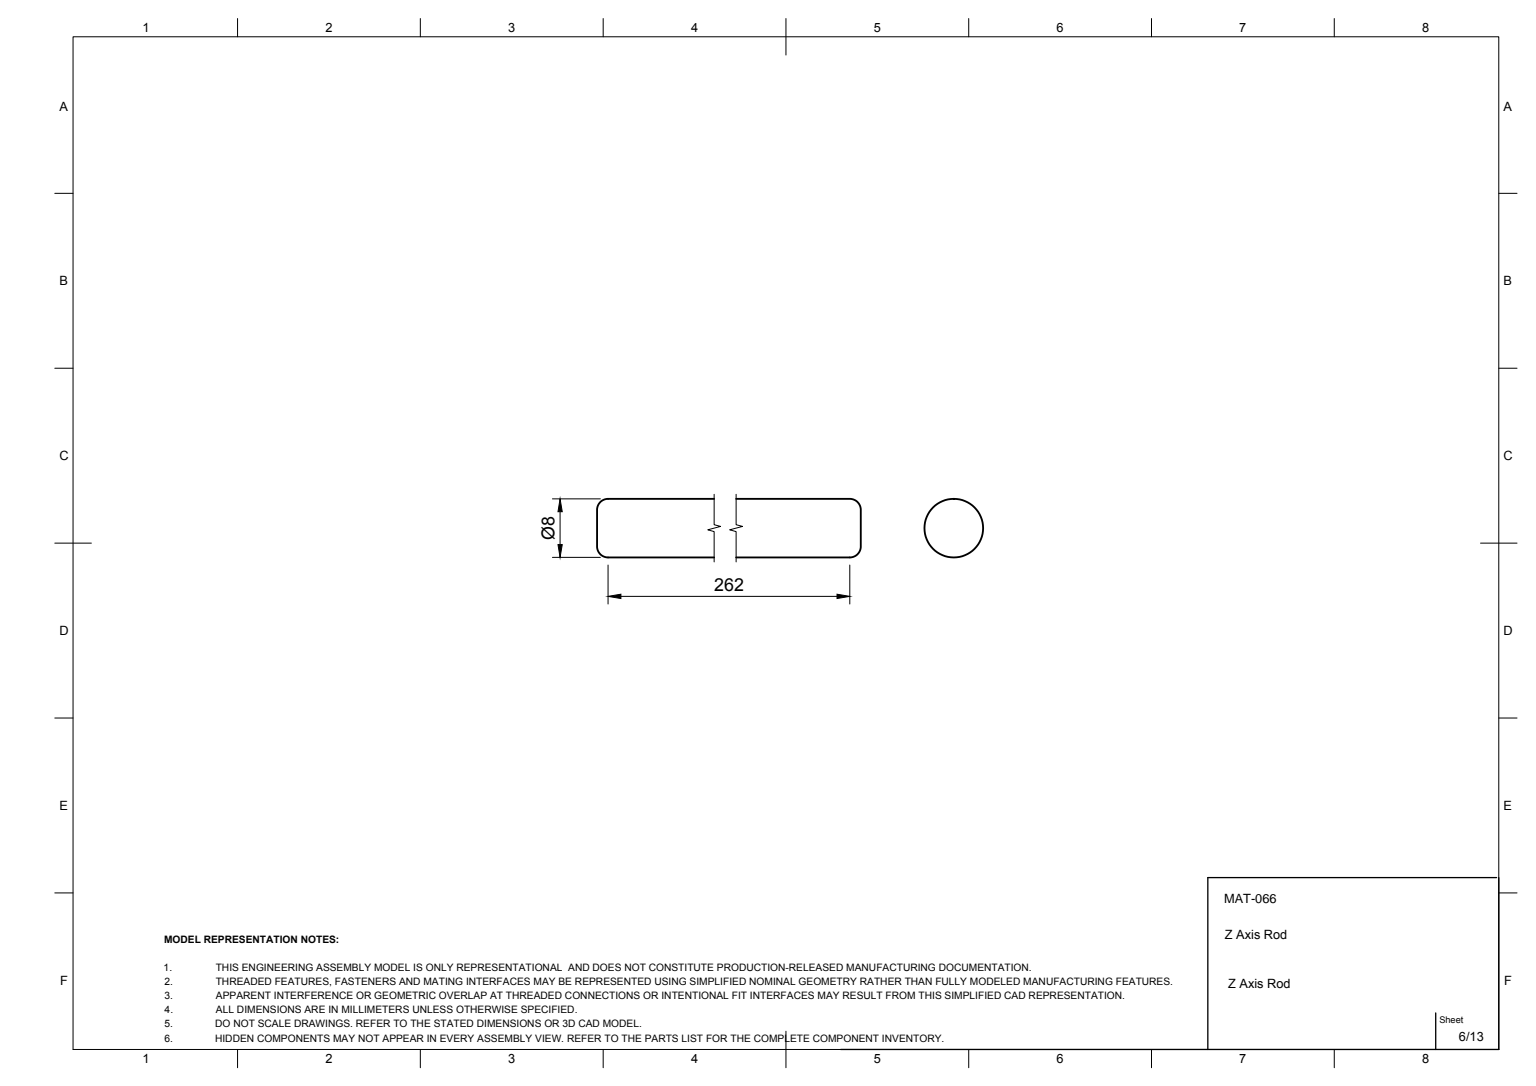
ISO-10303-21;
HEADER;
/* Generated by software containing ST-Developer
 * from STEP Tools, Inc. (www.steptools.com) 
 */

FILE_DESCRIPTION(
/* description */ ('CAx-IF Rec.Pracs.---Representation and Presentation of Product Manufa
cturing Information (PMI)---4.0---2014-10-13'),
/* implementation_level */ '2;1');

FILE_NAME(
/* name */ 'Z Axis Rod.step',
/* time_stamp */ '2026-10-24T15:58:00-07:00',
/* author */ (''),
/* organization */ (''),
/* preprocessor_version */ 'ST-DEVELOPER v20.2',
/* originating_system */ 'Autodesk Translation Framework v15.17.0.0',
/* authorisation */ '');

FILE_SCHEMA (('AP242_MANAGED_MODEL_BASED_3D_ENGINEERING_MIM_LF { 1 0 10303 442 2 1 4 }'));
ENDSEC;

DATA;
#10=MECHANICAL_DESIGN_GEOMETRIC_PRESENTATION_REPRESENTATION('',(#132),#8944);
#109=TOROIDAL_SURFACE('',#5681,0.0025,0.0015);
#110=TOROIDAL_SURFACE('',#5683,0.0025,0.0015);
#114=SHAPE_REPRESENTATION_RELATIONSHIP('SRR','None',#8996,#123);
#123=ADVANCED_BREP_SHAPE_REPRESENTATION('',(#141),#8937);
#132=STYLED_ITEM('',(#9055),#141);
#141=MANIFOLD_SOLID_BREP('Body1',#5153);
#217=CYLINDRICAL_SURFACE('',#5672,0.004);
#522=FACE_OUTER_BOUND('',#841,.T.);
#523=FACE_OUTER_BOUND('',#842,.T.);
#524=FACE_OUTER_BOUND('',#843,.T.);
#525=FACE_OUTER_BOUND('',#844,.T.);
#526=FACE_OUTER_BOUND('',#845,.T.);
#841=EDGE_LOOP('',(#4523,#4524,#4525,#4526,#4527,#4528));
#842=EDGE_LOOP('',(#4529));
#843=EDGE_LOOP('',(#4530));
#844=EDGE_LOOP('',(#4531,#4532,#4533,#4534,#4535));
#845=EDGE_LOOP('',(#4536,#4537,#4538,#4539,#4540));
#1110=CIRCLE('',#5673,0.004);
#1111=CIRCLE('',#5674,0.004);
#1112=CIRCLE('',#5675,0.004);
#1113=CIRCLE('',#5676,0.004);
#1114=CIRCLE('',#5678,0.0025);
#1115=CIRCLE('',#5680,0.0025);
#1116=CIRCLE('',#5682,0.0015);
#1117=CIRCLE('',#5684,0.0015);
#1596=LINE('',#8690,#2051);
#2051=VECTOR('',#7071,0.004);
#2498=VERTEX_POINT('',#8686);
#2499=VERTEX_POINT('',#8687);
#2500=VERTEX_POINT('',#8689);
#2501=VERTEX_POINT('',#8691);
#2502=VERTEX_POINT('',#8696);
#2503=VERTEX_POINT('',#8699);
#3182=EDGE_CURVE('',#2498,#2499,#1110,.T.);
#3183=EDGE_CURVE('',#2499,#2500,#1596,.T.);
#3184=EDGE_CURVE('',#2500,#2501,#1111,.F.);
#3185=EDGE_CURVE('',#2501,#2500,#1112,.F.);
#3186=EDGE_CURVE('',#2499,#2498,#1113,.T.);
#3187=EDGE_CURVE('',#2502,#2502,#1114,.T.);
#3188=EDGE_CURVE('',#2503,#2503,#1115,.F.);
#3189=EDGE_CURVE('',#2498,#2503,#1116,.T.);
#3190=EDGE_CURVE('',#2502,#2501,#1117,.T.);
#4523=ORIENTED_EDGE('',*,*,#3182,.T.);
#4524=ORIENTED_EDGE('',*,*,#3183,.T.);
#4525=ORIENTED_EDGE('',*,*,#3184,.T.);
#4526=ORIENTED_EDGE('',*,*,#3185,.T.);
#4527=ORIENTED_EDGE('',*,*,#3183,.F.);
#4528=ORIENTED_EDGE('',*,*,#3186,.T.);
#4529=ORIENTED_EDGE('',*,*,#3187,.T.);
#4530=ORIENTED_EDGE('',*,*,#3188,.T.);
#4531=ORIENTED_EDGE('',*,*,#3182,.F.);
#4532=ORIENTED_EDGE('',*,*,#3189,.T.);
#4533=ORIENTED_EDGE('',*,*,#3188,.F.);
#4534=ORIENTED_EDGE('',*,*,#3189,.F.);
#4535=ORIENTED_EDGE('',*,*,#3186,.F.);
#4536=ORIENTED_EDGE('',*,*,#3187,.F.);
#4537=ORIENTED_EDGE('',*,*,#3190,.T.);
#4538=ORIENTED_EDGE('',*,*,#3184,.F.);
#4539=ORIENTED_EDGE('',*,*,#3185,.F.);
#4540=ORIENTED_EDGE('',*,*,#3190,.F.);
#4859=PLANE('',#5677);
#4860=PLANE('',#5679);
#5095=ADVANCED_FACE('',(#522),#217,.T.);
#5096=ADVANCED_FACE('',(#523),#4859,.T.);
#5097=ADVANCED_FACE('',(#524),#4860,.F.);
#5098=ADVANCED_FACE('',(#525),#109,.T.);
#5099=ADVANCED_FACE('',(#526),#110,.T.);
#5153=CLOSED_SHELL('',(#5095,#5096,#5097,#5098,#5099));
#5671=AXIS2_PLACEMENT_3D('',#8684,#7065,#7066);
#5672=AXIS2_PLACEMENT_3D('',#8685,#7067,#7068);
#5673=AXIS2_PLACEMENT_3D('',#8688,#7069,#7070);
#5674=AXIS2_PLACEMENT_3D('',#8692,#7072,#7073);
#5675=AXIS2_PLACEMENT_3D('',#8693,#7074,#7075);
#5676=AXIS2_PLACEMENT_3D('',#8694,#7076,#7077);
#5677=AXIS2_PLACEMENT_3D('',#8695,#7078,#7079);
#5678=AXIS2_PLACEMENT_3D('',#8697,#7080,#7081);
#5679=AXIS2_PLACEMENT_3D('',#8698,#7082,#7083);
#5680=AXIS2_PLACEMENT_3D('',#8700,#7084,#7085);
#5681=AXIS2_PLACEMENT_3D('',#8701,#7086,#7087);
#5682=AXIS2_PLACEMENT_3D('',#8702,#7088,#7089);
#5683=AXIS2_PLACEMENT_3D('',#8703,#7090,#7091);
#5684=AXIS2_PLACEMENT_3D('',#8704,#7092,#7093);
#7065=DIRECTION('axis',(0.,0.,1.));
#7066=DIRECTION('refdir',(1.,0.,0.));
#7067=DIRECTION('center_axis',(0.,0.,-1.));
#7068=DIRECTION('ref_axis',(-1.,0.,0.));
#7069=DIRECTION('center_axis',(0.,0.,1.));
#7070=DIRECTION('ref_axis',(1.,0.,0.));
#7071=DIRECTION('',(0.,0.,1.));
#7072=DIRECTION('center_axis',(0.,0.,1.));
#7073=DIRECTION('ref_axis',(1.,0.,0.));
#7074=DIRECTION('center_axis',(0.,0.,1.));
#7075=DIRECTION('ref_axis',(1.,0.,0.));
#7076=DIRECTION('center_axis',(0.,0.,1.));
#7077=DIRECTION('ref_axis',(1.,0.,0.));
#7078=DIRECTION('center_axis',(0.,0.,1.));
#7079=DIRECTION('ref_axis',(1.,0.,0.));
#7080=DIRECTION('center_axis',(0.,0.,1.));
#7081=DIRECTION('ref_axis',(1.,0.,0.));
#7082=DIRECTION('center_axis',(0.,0.,1.));
#7083=DIRECTION('ref_axis',(1.,0.,0.));
#7084=DIRECTION('center_axis',(0.,0.,1.));
#7085=DIRECTION('ref_axis',(1.,0.,0.));
#7086=DIRECTION('center_axis',(0.,0.,1.));
#7087=DIRECTION('ref_axis',(1.,0.,0.));
#7088=DIRECTION('center_axis',(1.22464679914735E-16,-1.,0.));
#7089=DIRECTION('ref_axis',(-1.,-1.22464679914735E-16,0.));
#7090=DIRECTION('center_axis',(0.,0.,1.));
#7091=DIRECTION('ref_axis',(1.,0.,0.));
#7092=DIRECTION('center_axis',(1.22464679914735E-16,-1.,0.));
#7093=DIRECTION('ref_axis',(-1.,-1.22464679914735E-16,0.));
#8684=CARTESIAN_POINT('',(0.,0.,0.));
#8685=CARTESIAN_POINT('Origin',(0.,2.4492935982947E-19,0.265));
#8686=CARTESIAN_POINT('',(-0.004,-2.44929359829471E-19,0.0015));
#8687=CARTESIAN_POINT('',(0.004,-2.44929359829471E-19,0.00149999999999999));
#8688=CARTESIAN_POINT('Origin',(0.,2.4492935982947E-19,0.0015));
#8689=CARTESIAN_POINT('',(0.004,-2.44929359829471E-19,0.2635));
#8690=CARTESIAN_POINT('',(0.004,-2.44929359829471E-19,0.265));
#8691=CARTESIAN_POINT('',(-0.004,-2.44929359829471E-19,0.2635));
#8692=CARTESIAN_POINT('Origin',(0.,2.4492935982947E-19,0.2635));
#8693=CARTESIAN_POINT('Origin',(0.,2.4492935982947E-19,0.2635));
#8694=CARTESIAN_POINT('Origin',(0.,2.4492935982947E-19,0.0015));
#8695=CARTESIAN_POINT('Origin',(0.,0.,0.265));
#8696=CARTESIAN_POINT('',(-0.0025,-6.12323399573683E-20,0.265));
#8697=CARTESIAN_POINT('Origin',(0.,2.4492935982947E-19,0.265));
#8698=CARTESIAN_POINT('Origin',(0.,0.,0.));
#8699=CARTESIAN_POINT('',(-0.0025,-6.12323399573683E-20,0.));
#8700=CARTESIAN_POINT('Origin',(0.,2.4492935982947E-19,0.));
#8701=CARTESIAN_POINT('Origin',(0.,2.4492935982947E-19,0.0015));
#8702=CARTESIAN_POINT('Origin',(-0.0025,-6.12323399573683E-20,0.0015));
#8703=CARTESIAN_POINT('Origin',(0.,2.4492935982947E-19,0.2635));
#8704=CARTESIAN_POINT('Origin',(-0.0025,-6.12323399573683E-20,0.2635));
#8925=UNCERTAINTY_MEASURE_WITH_UNIT(LENGTH_MEASURE(1.E-5),#8945,
'DISTANCE_ACCURACY_VALUE',
'Maximum model space distance between geometric entities at asserted c
onnectivities');
#8932=UNCERTAINTY_MEASURE_WITH_UNIT(LENGTH_MEASURE(1.E-5),#8945,
'DISTANCE_ACCURACY_VALUE',
'Maximum model space distance between geometric entities at asserted c
onnectivities');
#8937=(
GEOMETRIC_REPRESENTATION_CONTEXT(3)
GLOBAL_UNCERTAINTY_ASSIGNED_CONTEXT((#8925))
GLOBAL_UNIT_ASSIGNED_CONTEXT((#8945,#8946,#8947))
REPRESENTATION_CONTEXT('','3D')
);
#8944=(
GEOMETRIC_REPRESENTATION_CONTEXT(3)
GLOBAL_UNCERTAINTY_ASSIGNED_CONTEXT((#8932))
GLOBAL_UNIT_ASSIGNED_CONTEXT((#8945,#8946,#8947))
REPRESENTATION_CONTEXT('','3D')
);
#8945=(
LENGTH_UNIT()
NAMED_UNIT(*)
SI_UNIT($,.METRE.)
);
#8946=(
NAMED_UNIT(*)
PLANE_ANGLE_UNIT()
SI_UNIT($,.RADIAN.)
);
#8947=(
NAMED_UNIT(*)
SI_UNIT($,.STERADIAN.)
SOLID_ANGLE_UNIT()
);
#8952=SHAPE_DEFINITION_REPRESENTATION(#8963,#8996);
#8963=PRODUCT_DEFINITION_SHAPE('',$,#9008);
#8996=SHAPE_REPRESENTATION('',(#5671),#8937);
#9003=PRODUCT_DEFINITION_CONTEXT('part definition',#9038,'design');
#9008=PRODUCT_DEFINITION('Z Axis Rod','Z Axis Rod',#9019,#9003);
#9019=PRODUCT_DEFINITION_FORMATION('',$,#9044);
#9038=APPLICATION_CONTEXT('Managed model based 3d engineering');
#9039=PRODUCT_CONTEXT('part definition',#9038,'mechanical');
#9044=PRODUCT('Z Axis Rod','Z Axis Rod',
'LEGAL AND USAGE DISCLAIMER: this Data/Model is provided \X2\201C\X0\A
S IS\X2\201D\X0\ for informational and representational only. It is a 
geometric approximation and is NOT engineered, certified, or guarantee
d for dimensional accuracy, exact tolerances, or production-level prec
ision. Vendor disclaims all implied warranties including fitness for a
 particular purpose. DO NOT USE FOR DIRECT PHYSICAL MANUFACTURING, AUT
OMATED PRODUCTION, OR SAFETY-CRITICAL SYSTEMS without independent engi
neering verification and resolution of any design discrepancies.',(#9039));
#9055=PRESENTATION_STYLE_ASSIGNMENT((#9060));
#9060=SURFACE_STYLE_USAGE(.BOTH.,#9065);
#9065=SURFACE_SIDE_STYLE('',(#9070));
#9070=SURFACE_STYLE_FILL_AREA(#9075);
#9075=FILL_AREA_STYLE('Opaque(48,59,150)',(#9080));
#9080=FILL_AREA_STYLE_COLOUR('Opaque(48,59,150)',#9085);
#9085=COLOUR_RGB('Opaque(48,59,150)',0.188235294117647,0.231372549019608,
0.588235294117647);
ENDSEC;
END-ISO-10303-21;
